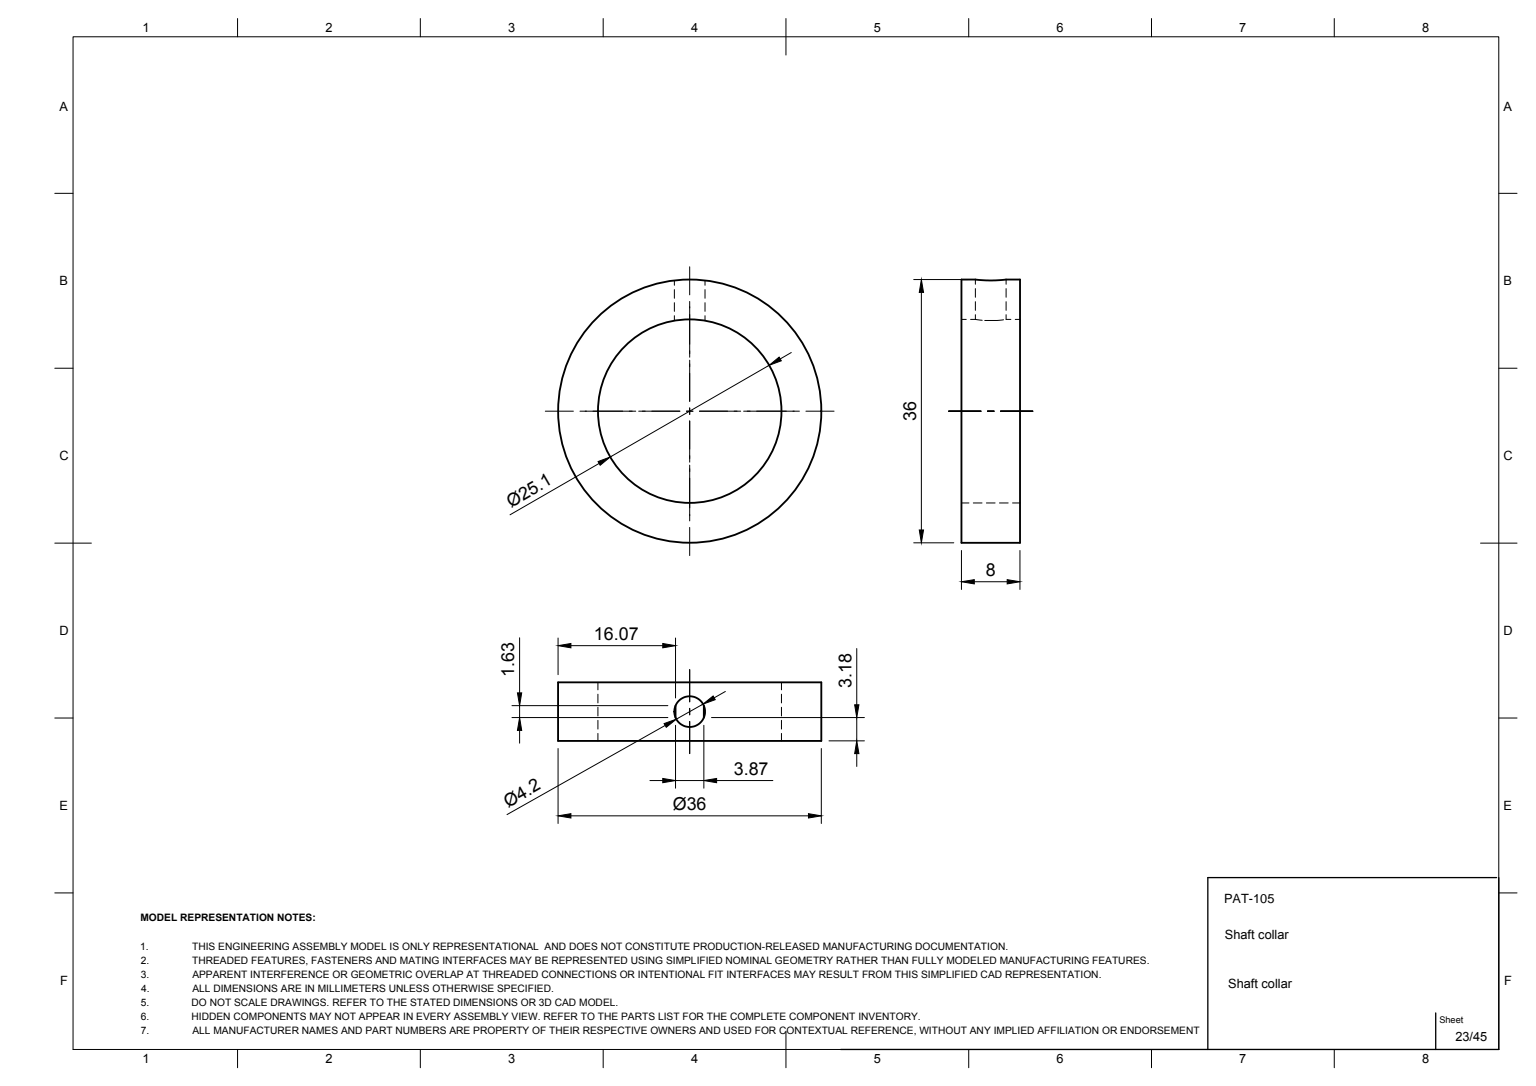
ISO-10303-21;
HEADER;
/* Generated by software containing ST-Developer
 * from STEP Tools, Inc. (www.steptools.com) 
 */

FILE_DESCRIPTION(
/* description */ ('Torque wrench calibration arm'),
/* implementation_level */ '2;1');

FILE_NAME(
/* name */ 'Shaft collar.step',
/* time_stamp */ '2026-10-28T03:24:52-07:00',
/* author */ (''),
/* organization */ (''),
/* preprocessor_version */ 'ST-DEVELOPER v20.2',
/* originating_system */ 'Autodesk Translation Framework v15.17.0.0',
/* authorisation */ '');

FILE_SCHEMA (('AUTOMOTIVE_DESIGN { 1 0 10303 214 3 1 1 }'));
ENDSEC;

DATA;
#10=MECHANICAL_DESIGN_GEOMETRIC_PRESENTATION_REPRESENTATION('',(#451),#12783);
#263=B_SPLINE_CURVE_WITH_KNOTS('',3,(#11304,#11305,#11306,#11307,#11308,
#11309,#11310,#11311,#11312,#11313,#11314,#11315,#11316,#11317),
 .UNSPECIFIED.,.F.,.F.,(4,2,2,2,2,2,4),(0.714680326757342,0.79264866270072,
0.871912238073927,0.951175813447134,1.03043938882034,1.10970296419355,1.18767130013693),
 .UNSPECIFIED.);
#264=B_SPLINE_CURVE_WITH_KNOTS('',3,(#11323,#11324,#11325,#11326,#11327,
#11328,#11329,#11330,#11331,#11332,#11333,#11334,#11335,#11336,#11337,#11338,
#11339,#11340),.UNSPECIFIED.,.F.,.F.,(4,2,2,2,2,2,2,2,4),(0.,0.0791819055472369,
0.158363811094474,0.237545215630596,0.316726620166718,0.395908024702839,
0.475089429238961,0.554271334786198,0.633453240333435),.UNSPECIFIED.);
#265=B_SPLINE_CURVE_WITH_KNOTS('',3,(#11341,#11342,#11343,#11344,#11345,
#11346,#11347,#11348,#11349,#11350,#11351,#11352,#11353,#11354,#11355,#11356,
#11357,#11358),.UNSPECIFIED.,.F.,.F.,(4,2,2,2,2,2,2,2,4),(0.633453240333435,
0.712635145880672,0.791817051427908,0.87099845596403,0.950179860500152,
1.02936126503627,1.1085426695724,1.18772457511963,1.26690648066687),
 .UNSPECIFIED.);
#266=B_SPLINE_CURVE_WITH_KNOTS('',3,(#11361,#11362,#11363,#11364,#11365,
#11366,#11367,#11368,#11369,#11370,#11371,#11372,#11373,#11374),
 .UNSPECIFIED.,.F.,.F.,(4,2,2,2,2,2,4),(0.080563117792587,0.158531453735964,
0.237795029109171,0.317058604482378,0.396322179855585,0.475585755228792,
0.553554091172169),.UNSPECIFIED.);
#368=SHAPE_REPRESENTATION_RELATIONSHIP('SRR','None',#12951,#405);
#405=ADVANCED_BREP_SHAPE_REPRESENTATION('',(#503),#12760);
#451=STYLED_ITEM('',(#13212),#503);
#503=MANIFOLD_SOLID_BREP('Body1',#6522);
#600=FACE_BOUND('',#1552,.T.);
#601=FACE_BOUND('',#1554,.T.);
#602=FACE_BOUND('',#1556,.T.);
#603=FACE_BOUND('',#1558,.T.);
#766=PLANE('',#7413);
#767=PLANE('',#7418);
#768=PLANE('',#7425);
#769=PLANE('',#7426);
#1084=FACE_OUTER_BOUND('',#1548,.T.);
#1085=FACE_OUTER_BOUND('',#1549,.T.);
#1086=FACE_OUTER_BOUND('',#1550,.T.);
#1087=FACE_OUTER_BOUND('',#1551,.T.);
#1088=FACE_OUTER_BOUND('',#1553,.T.);
#1089=FACE_OUTER_BOUND('',#1555,.T.);
#1090=FACE_OUTER_BOUND('',#1557,.T.);
#1548=EDGE_LOOP('',(#5227,#5228));
#1549=EDGE_LOOP('',(#5229,#5230,#5231,#5232,#5233,#5234,#5235,#5236,#5237));
#1550=EDGE_LOOP('',(#5238,#5239,#5240));
#1551=EDGE_LOOP('',(#5241,#5242,#5243,#5244));
#1552=EDGE_LOOP('',(#5245,#5246,#5247,#5248));
#1553=EDGE_LOOP('',(#5249,#5250,#5251,#5252));
#1554=EDGE_LOOP('',(#5253,#5254));
#1555=EDGE_LOOP('',(#5255));
#1556=EDGE_LOOP('',(#5256));
#1557=EDGE_LOOP('',(#5257));
#1558=EDGE_LOOP('',(#5258));
#2009=LINE('',#11300,#2424);
#2010=LINE('',#11321,#2425);
#2011=LINE('',#11376,#2426);
#2012=LINE('',#11381,#2427);
#2013=LINE('',#11387,#2428);
#2424=VECTOR('',#8941,1.);
#2425=VECTOR('',#8948,0.21);
#2426=VECTOR('',#8953,1.);
#2427=VECTOR('',#8958,1.255);
#2428=VECTOR('',#8965,1.8);
#2813=CIRCLE('',#7414,0.21);
#2814=CIRCLE('',#7416,0.21);
#2815=CIRCLE('',#7417,0.21);
#2816=CIRCLE('',#7420,1.255);
#2817=CIRCLE('',#7421,1.255);
#2818=CIRCLE('',#7423,1.8);
#2819=CIRCLE('',#7424,1.8);
#3271=VERTEX_POINT('',#11298);
#3272=VERTEX_POINT('',#11299);
#3273=VERTEX_POINT('',#11303);
#3274=VERTEX_POINT('',#11318);
#3275=VERTEX_POINT('',#11320);
#3276=VERTEX_POINT('',#11322);
#3277=VERTEX_POINT('',#11359);
#3278=VERTEX_POINT('',#11378);
#3279=VERTEX_POINT('',#11380);
#3280=VERTEX_POINT('',#11384);
#3281=VERTEX_POINT('',#11386);
#3971=EDGE_CURVE('',#3271,#3272,#2009,.T.);
#3972=EDGE_CURVE('',#3271,#3272,#2813,.T.);
#3973=EDGE_CURVE('',#3273,#3271,#263,.T.);
#3974=EDGE_CURVE('',#3274,#3273,#2814,.T.);
#3975=EDGE_CURVE('',#3274,#3275,#2010,.T.);
#3976=EDGE_CURVE('',#3276,#3275,#264,.T.);
#3977=EDGE_CURVE('',#3275,#3276,#265,.T.);
#3978=EDGE_CURVE('',#3277,#3274,#2815,.T.);
#3979=EDGE_CURVE('',#3272,#3277,#266,.T.);
#3980=EDGE_CURVE('',#3277,#3273,#2011,.T.);
#3981=EDGE_CURVE('',#3278,#3278,#2816,.T.);
#3982=EDGE_CURVE('',#3278,#3279,#2012,.T.);
#3983=EDGE_CURVE('',#3279,#3279,#2817,.T.);
#3984=EDGE_CURVE('',#3280,#3280,#2818,.T.);
#3985=EDGE_CURVE('',#3280,#3281,#2013,.T.);
#3986=EDGE_CURVE('',#3281,#3281,#2819,.T.);
#5227=ORIENTED_EDGE('',*,*,#3971,.F.);
#5228=ORIENTED_EDGE('',*,*,#3972,.T.);
#5229=ORIENTED_EDGE('',*,*,#3973,.F.);
#5230=ORIENTED_EDGE('',*,*,#3974,.F.);
#5231=ORIENTED_EDGE('',*,*,#3975,.T.);
#5232=ORIENTED_EDGE('',*,*,#3976,.F.);
#5233=ORIENTED_EDGE('',*,*,#3977,.F.);
#5234=ORIENTED_EDGE('',*,*,#3975,.F.);
#5235=ORIENTED_EDGE('',*,*,#3978,.F.);
#5236=ORIENTED_EDGE('',*,*,#3979,.F.);
#5237=ORIENTED_EDGE('',*,*,#3972,.F.);
#5238=ORIENTED_EDGE('',*,*,#3980,.F.);
#5239=ORIENTED_EDGE('',*,*,#3978,.T.);
#5240=ORIENTED_EDGE('',*,*,#3974,.T.);
#5241=ORIENTED_EDGE('',*,*,#3981,.F.);
#5242=ORIENTED_EDGE('',*,*,#3982,.T.);
#5243=ORIENTED_EDGE('',*,*,#3983,.T.);
#5244=ORIENTED_EDGE('',*,*,#3982,.F.);
#5245=ORIENTED_EDGE('',*,*,#3979,.T.);
#5246=ORIENTED_EDGE('',*,*,#3980,.T.);
#5247=ORIENTED_EDGE('',*,*,#3973,.T.);
#5248=ORIENTED_EDGE('',*,*,#3971,.T.);
#5249=ORIENTED_EDGE('',*,*,#3984,.F.);
#5250=ORIENTED_EDGE('',*,*,#3985,.T.);
#5251=ORIENTED_EDGE('',*,*,#3986,.T.);
#5252=ORIENTED_EDGE('',*,*,#3985,.F.);
#5253=ORIENTED_EDGE('',*,*,#3976,.T.);
#5254=ORIENTED_EDGE('',*,*,#3977,.T.);
#5255=ORIENTED_EDGE('',*,*,#3984,.T.);
#5256=ORIENTED_EDGE('',*,*,#3981,.T.);
#5257=ORIENTED_EDGE('',*,*,#3986,.F.);
#5258=ORIENTED_EDGE('',*,*,#3983,.F.);
#6050=CYLINDRICAL_SURFACE('',#7415,0.21);
#6051=CYLINDRICAL_SURFACE('',#7419,1.255);
#6052=CYLINDRICAL_SURFACE('',#7422,1.8);
#6309=ADVANCED_FACE('',(#1084),#766,.T.);
#6310=ADVANCED_FACE('',(#1085),#6050,.F.);
#6311=ADVANCED_FACE('',(#1086),#767,.T.);
#6312=ADVANCED_FACE('',(#1087,#600),#6051,.F.);
#6313=ADVANCED_FACE('',(#1088,#601),#6052,.T.);
#6314=ADVANCED_FACE('',(#1089,#602),#768,.T.);
#6315=ADVANCED_FACE('',(#1090,#603),#769,.F.);
#6522=CLOSED_SHELL('',(#6309,#6310,#6311,#6312,#6313,#6314,#6315));
#7412=AXIS2_PLACEMENT_3D('',#11296,#8937,#8938);
#7413=AXIS2_PLACEMENT_3D('',#11297,#8939,#8940);
#7414=AXIS2_PLACEMENT_3D('',#11301,#8942,#8943);
#7415=AXIS2_PLACEMENT_3D('',#11302,#8944,#8945);
#7416=AXIS2_PLACEMENT_3D('',#11319,#8946,#8947);
#7417=AXIS2_PLACEMENT_3D('',#11360,#8949,#8950);
#7418=AXIS2_PLACEMENT_3D('',#11375,#8951,#8952);
#7419=AXIS2_PLACEMENT_3D('',#11377,#8954,#8955);
#7420=AXIS2_PLACEMENT_3D('',#11379,#8956,#8957);
#7421=AXIS2_PLACEMENT_3D('',#11382,#8959,#8960);
#7422=AXIS2_PLACEMENT_3D('',#11383,#8961,#8962);
#7423=AXIS2_PLACEMENT_3D('',#11385,#8963,#8964);
#7424=AXIS2_PLACEMENT_3D('',#11388,#8966,#8967);
#7425=AXIS2_PLACEMENT_3D('',#11389,#8968,#8969);
#7426=AXIS2_PLACEMENT_3D('',#11390,#8970,#8971);
#8937=DIRECTION('axis',(0.,0.,1.));
#8938=DIRECTION('refdir',(1.,0.,0.));
#8939=DIRECTION('center_axis',(0.,0.,1.));
#8940=DIRECTION('ref_axis',(1.,0.,0.));
#8941=DIRECTION('',(0.,1.,0.));
#8942=DIRECTION('center_axis',(0.,0.,1.));
#8943=DIRECTION('ref_axis',(1.,0.,0.));
#8944=DIRECTION('center_axis',(0.,0.,1.));
#8945=DIRECTION('ref_axis',(1.,0.,0.));
#8946=DIRECTION('center_axis',(0.,0.,1.));
#8947=DIRECTION('ref_axis',(1.,0.,0.));
#8948=DIRECTION('',(0.,0.,1.));
#8949=DIRECTION('center_axis',(0.,0.,1.));
#8950=DIRECTION('ref_axis',(1.,0.,0.));
#8951=DIRECTION('center_axis',(0.,0.,1.));
#8952=DIRECTION('ref_axis',(1.,0.,0.));
#8953=DIRECTION('',(0.,-1.,0.));
#8954=DIRECTION('center_axis',(0.,1.,0.));
#8955=DIRECTION('ref_axis',(1.,0.,0.));
#8956=DIRECTION('center_axis',(0.,-1.,0.));
#8957=DIRECTION('ref_axis',(1.,0.,0.));
#8958=DIRECTION('',(0.,-1.,0.));
#8959=DIRECTION('center_axis',(0.,-1.,0.));
#8960=DIRECTION('ref_axis',(1.,0.,0.));
#8961=DIRECTION('center_axis',(0.,1.,0.));
#8962=DIRECTION('ref_axis',(1.,0.,0.));
#8963=DIRECTION('center_axis',(0.,1.,0.));
#8964=DIRECTION('ref_axis',(1.,0.,0.));
#8965=DIRECTION('',(0.,-1.,0.));
#8966=DIRECTION('center_axis',(0.,1.,0.));
#8967=DIRECTION('ref_axis',(1.,0.,0.));
#8968=DIRECTION('center_axis',(0.,1.,0.));
#8969=DIRECTION('ref_axis',(1.,0.,0.));
#8970=DIRECTION('center_axis',(0.,1.,0.));
#8971=DIRECTION('ref_axis',(1.,0.,0.));
#11296=CARTESIAN_POINT('',(0.,0.,0.));
#11297=CARTESIAN_POINT('Origin',(0.,6.8,9.24));
#11298=CARTESIAN_POINT('',(0.193455421221531,6.71829932680816,9.24));
#11299=CARTESIAN_POINT('',(0.193455421221531,6.88170067319184,9.24));
#11300=CARTESIAN_POINT('',(0.193455421221531,6.4,9.24));
#11301=CARTESIAN_POINT('Origin',(0.,6.8,9.24));
#11302=CARTESIAN_POINT('Origin',(0.,6.8,9.24));
#11303=CARTESIAN_POINT('',(-0.193455421221531,6.71829932680816,9.24));
#11304=CARTESIAN_POINT('Ctrl Pts',(-0.193455421221531,6.71829932680816,
9.24));
#11305=CARTESIAN_POINT('Ctrl Pts',(-0.182741806873435,6.69293103184137,
9.24167145707784));
#11306=CARTESIAN_POINT('Ctrl Pts',(-0.166804849537961,6.66982000143961,
9.24400210952839));
#11307=CARTESIAN_POINT('Ctrl Pts',(-0.129875785635207,6.63289093753686,
9.24840249136865));
#11308=CARTESIAN_POINT('Ctrl Pts',(-0.106295060941802,6.6167372734261,9.2507589672592));
#11309=CARTESIAN_POINT('Ctrl Pts',(-0.0545698089447934,6.59529044194989,
9.25408084670822));
#11310=CARTESIAN_POINT('Ctrl Pts',(-0.0264211917910691,6.59,9.255));
#11311=CARTESIAN_POINT('Ctrl Pts',(0.026421191791069,6.59,9.255));
#11312=CARTESIAN_POINT('Ctrl Pts',(0.0545698089447934,6.59529044194989,
9.25408084670822));
#11313=CARTESIAN_POINT('Ctrl Pts',(0.106295060941802,6.6167372734261,9.2507589672592));
#11314=CARTESIAN_POINT('Ctrl Pts',(0.129875785635207,6.63289093753686,9.24840249136865));
#11315=CARTESIAN_POINT('Ctrl Pts',(0.166804849537961,6.66982000143961,9.24400210952839));
#11316=CARTESIAN_POINT('Ctrl Pts',(0.182741806873435,6.69293103184137,9.24167145707784));
#11317=CARTESIAN_POINT('Ctrl Pts',(0.193455421221531,6.71829932680816,9.24));
#11318=CARTESIAN_POINT('',(-0.21,6.8,9.24));
#11319=CARTESIAN_POINT('Origin',(0.,6.8,9.24));
#11320=CARTESIAN_POINT('',(-0.21,6.8,9.78770802985275));
#11321=CARTESIAN_POINT('',(-0.21,6.8,9.24));
#11322=CARTESIAN_POINT('',(0.21,6.8,9.78770802985275));
#11323=CARTESIAN_POINT('Ctrl Pts',(0.21,6.8,9.78770802985275));
#11324=CARTESIAN_POINT('Ctrl Pts',(0.21,6.77360603148425,9.78770802985275));
#11325=CARTESIAN_POINT('Ctrl Pts',(0.204720232951726,6.74546934556601,9.78835284034214));
#11326=CARTESIAN_POINT('Ctrl Pts',(0.183281523978899,6.69373688397397,9.79067700538683));
#11327=CARTESIAN_POINT('Ctrl Pts',(0.167123888882363,6.67013904078401,9.79232226897314));
#11328=CARTESIAN_POINT('Ctrl Pts',(0.129861077103665,6.63287622900531,9.79540680803063));
#11329=CARTESIAN_POINT('Ctrl Pts',(0.106263182528071,6.6167185016358,9.79704717240673));
#11330=CARTESIAN_POINT('Ctrl Pts',(0.0545305475112071,6.59527972468261,
9.79936011492601));
#11331=CARTESIAN_POINT('Ctrl Pts',(0.0263938015120406,6.59,9.8));
#11332=CARTESIAN_POINT('Ctrl Pts',(-0.0263938015120406,6.59,9.8));
#11333=CARTESIAN_POINT('Ctrl Pts',(-0.054530547511207,6.59527972468261,
9.79936011492601));
#11334=CARTESIAN_POINT('Ctrl Pts',(-0.106263182528071,6.6167185016358,9.79704717240673));
#11335=CARTESIAN_POINT('Ctrl Pts',(-0.129861077103665,6.63287622900531,
9.79540680803063));
#11336=CARTESIAN_POINT('Ctrl Pts',(-0.167123888882363,6.67013904078401,
9.79232226897314));
#11337=CARTESIAN_POINT('Ctrl Pts',(-0.183281523978899,6.69373688397397,
9.79067700538683));
#11338=CARTESIAN_POINT('Ctrl Pts',(-0.204720232951726,6.74546934556601,
9.78835284034214));
#11339=CARTESIAN_POINT('Ctrl Pts',(-0.21,6.77360603148425,9.78770802985275));
#11340=CARTESIAN_POINT('Ctrl Pts',(-0.21,6.8,9.78770802985275));
#11341=CARTESIAN_POINT('Ctrl Pts',(-0.21,6.8,9.78770802985275));
#11342=CARTESIAN_POINT('Ctrl Pts',(-0.21,6.82639396851575,9.78770802985275));
#11343=CARTESIAN_POINT('Ctrl Pts',(-0.204720232951726,6.85453065443398,
9.78835284034214));
#11344=CARTESIAN_POINT('Ctrl Pts',(-0.1832815239789,6.90626311602603,9.79067700538683));
#11345=CARTESIAN_POINT('Ctrl Pts',(-0.167123888882363,6.92986095921599,
9.79232226897314));
#11346=CARTESIAN_POINT('Ctrl Pts',(-0.129861077103665,6.96712377099468,
9.79540680803063));
#11347=CARTESIAN_POINT('Ctrl Pts',(-0.106263182528071,6.9832814983642,9.79704717240673));
#11348=CARTESIAN_POINT('Ctrl Pts',(-0.0545305475112072,7.00472027531739,
9.79936011492601));
#11349=CARTESIAN_POINT('Ctrl Pts',(-0.0263938015120407,7.01,9.8));
#11350=CARTESIAN_POINT('Ctrl Pts',(0.0263938015120407,7.01,9.8));
#11351=CARTESIAN_POINT('Ctrl Pts',(0.0545305475112071,7.00472027531739,
9.79936011492601));
#11352=CARTESIAN_POINT('Ctrl Pts',(0.106263182528071,6.9832814983642,9.79704717240673));
#11353=CARTESIAN_POINT('Ctrl Pts',(0.129861077103665,6.96712377099468,9.79540680803063));
#11354=CARTESIAN_POINT('Ctrl Pts',(0.167123888882363,6.92986095921599,9.79232226897314));
#11355=CARTESIAN_POINT('Ctrl Pts',(0.1832815239789,6.90626311602603,9.79067700538683));
#11356=CARTESIAN_POINT('Ctrl Pts',(0.204720232951726,6.85453065443398,9.78835284034214));
#11357=CARTESIAN_POINT('Ctrl Pts',(0.21,6.82639396851575,9.78770802985275));
#11358=CARTESIAN_POINT('Ctrl Pts',(0.21,6.8,9.78770802985275));
#11359=CARTESIAN_POINT('',(-0.193455421221531,6.88170067319184,9.24));
#11360=CARTESIAN_POINT('Origin',(0.,6.8,9.24));
#11361=CARTESIAN_POINT('Ctrl Pts',(0.19345542122153,6.88170067319184,9.24));
#11362=CARTESIAN_POINT('Ctrl Pts',(0.182741806873435,6.90706896815863,9.24167145707784));
#11363=CARTESIAN_POINT('Ctrl Pts',(0.166804849537961,6.93017999856039,9.24400210952839));
#11364=CARTESIAN_POINT('Ctrl Pts',(0.129875785635207,6.96710906246314,9.24840249136865));
#11365=CARTESIAN_POINT('Ctrl Pts',(0.106295060941802,6.9832627265739,9.2507589672592));
#11366=CARTESIAN_POINT('Ctrl Pts',(0.0545698089447934,7.0047095580501,9.25408084670822));
#11367=CARTESIAN_POINT('Ctrl Pts',(0.026421191791069,7.01,9.255));
#11368=CARTESIAN_POINT('Ctrl Pts',(-0.026421191791069,7.01,9.255));
#11369=CARTESIAN_POINT('Ctrl Pts',(-0.0545698089447934,7.0047095580501,
9.25408084670822));
#11370=CARTESIAN_POINT('Ctrl Pts',(-0.106295060941802,6.9832627265739,9.2507589672592));
#11371=CARTESIAN_POINT('Ctrl Pts',(-0.129875785635207,6.96710906246314,
9.24840249136865));
#11372=CARTESIAN_POINT('Ctrl Pts',(-0.166804849537961,6.93017999856039,
9.24400210952839));
#11373=CARTESIAN_POINT('Ctrl Pts',(-0.182741806873435,6.90706896815863,
9.24167145707784));
#11374=CARTESIAN_POINT('Ctrl Pts',(-0.19345542122153,6.88170067319184,9.24));
#11375=CARTESIAN_POINT('Origin',(0.,6.8,9.24));
#11376=CARTESIAN_POINT('',(-0.193455421221531,6.4,9.24));
#11377=CARTESIAN_POINT('Origin',(0.,6.4,8.));
#11378=CARTESIAN_POINT('',(-1.255,7.2,8.));
#11379=CARTESIAN_POINT('Origin',(0.,7.2,8.));
#11380=CARTESIAN_POINT('',(-1.255,6.4,8.));
#11381=CARTESIAN_POINT('',(-1.255,6.4,8.));
#11382=CARTESIAN_POINT('Origin',(0.,6.4,8.));
#11383=CARTESIAN_POINT('Origin',(0.,6.4,8.));
#11384=CARTESIAN_POINT('',(-1.8,7.2,8.));
#11385=CARTESIAN_POINT('Origin',(0.,7.2,8.));
#11386=CARTESIAN_POINT('',(-1.8,6.4,8.));
#11387=CARTESIAN_POINT('',(-1.8,6.4,8.));
#11388=CARTESIAN_POINT('Origin',(0.,6.4,8.));
#11389=CARTESIAN_POINT('Origin',(0.,7.2,8.));
#11390=CARTESIAN_POINT('Origin',(0.,6.4,8.));
#12716=UNCERTAINTY_MEASURE_WITH_UNIT(LENGTH_MEASURE(0.001),#12784,
'DISTANCE_ACCURACY_VALUE',
'Maximum model space distance between geometric entities at asserted c
onnectivities');
#12739=UNCERTAINTY_MEASURE_WITH_UNIT(LENGTH_MEASURE(0.001),#12784,
'DISTANCE_ACCURACY_VALUE',
'Maximum model space distance between geometric entities at asserted c
onnectivities');
#12760=(
GEOMETRIC_REPRESENTATION_CONTEXT(3)
GLOBAL_UNCERTAINTY_ASSIGNED_CONTEXT((#12716))
GLOBAL_UNIT_ASSIGNED_CONTEXT((#12784,#12786,#12787))
REPRESENTATION_CONTEXT('','3D')
);
#12783=(
GEOMETRIC_REPRESENTATION_CONTEXT(3)
GLOBAL_UNCERTAINTY_ASSIGNED_CONTEXT((#12739))
GLOBAL_UNIT_ASSIGNED_CONTEXT((#12784,#12786,#12787))
REPRESENTATION_CONTEXT('','3D')
);
#12784=(
LENGTH_UNIT()
NAMED_UNIT(*)
SI_UNIT(.CENTI.,.METRE.)
);
#12786=(
NAMED_UNIT(*)
PLANE_ANGLE_UNIT()
SI_UNIT($,.RADIAN.)
);
#12787=(
NAMED_UNIT(*)
SI_UNIT($,.STERADIAN.)
SOLID_ANGLE_UNIT()
);
#12808=SHAPE_DEFINITION_REPRESENTATION(#12877,#12951);
#12877=PRODUCT_DEFINITION_SHAPE('',$,#12995);
#12951=SHAPE_REPRESENTATION('',(#7412),#12760);
#12974=PRODUCT_DEFINITION_CONTEXT('part definition',#13105,'design');
#12995=PRODUCT_DEFINITION('Shaft collar','Shaft collar',#13038,#12974);
#13038=PRODUCT_DEFINITION_FORMATION('',$,#13127);
#13105=APPLICATION_CONTEXT(
'Core Data for Automotive Mechanical Design Process');
#13106=PRODUCT_CONTEXT('part definition',#13105,'mechanical');
#13127=PRODUCT('Shaft collar','Shaft collar','Shaft collar',(#13106));
#13206=COLOUR_RGB('Grey',0.48,0.52,0.57);
#13207=FILL_AREA_STYLE_COLOUR('',#13206);
#13208=FILL_AREA_STYLE('',(#13207));
#13209=SURFACE_STYLE_FILL_AREA(#13208);
#13210=SURFACE_SIDE_STYLE('',(#13209));
#13211=SURFACE_STYLE_USAGE(.BOTH.,#13210);
#13212=PRESENTATION_STYLE_ASSIGNMENT((#13211));
ENDSEC;
END-ISO-10303-21;
